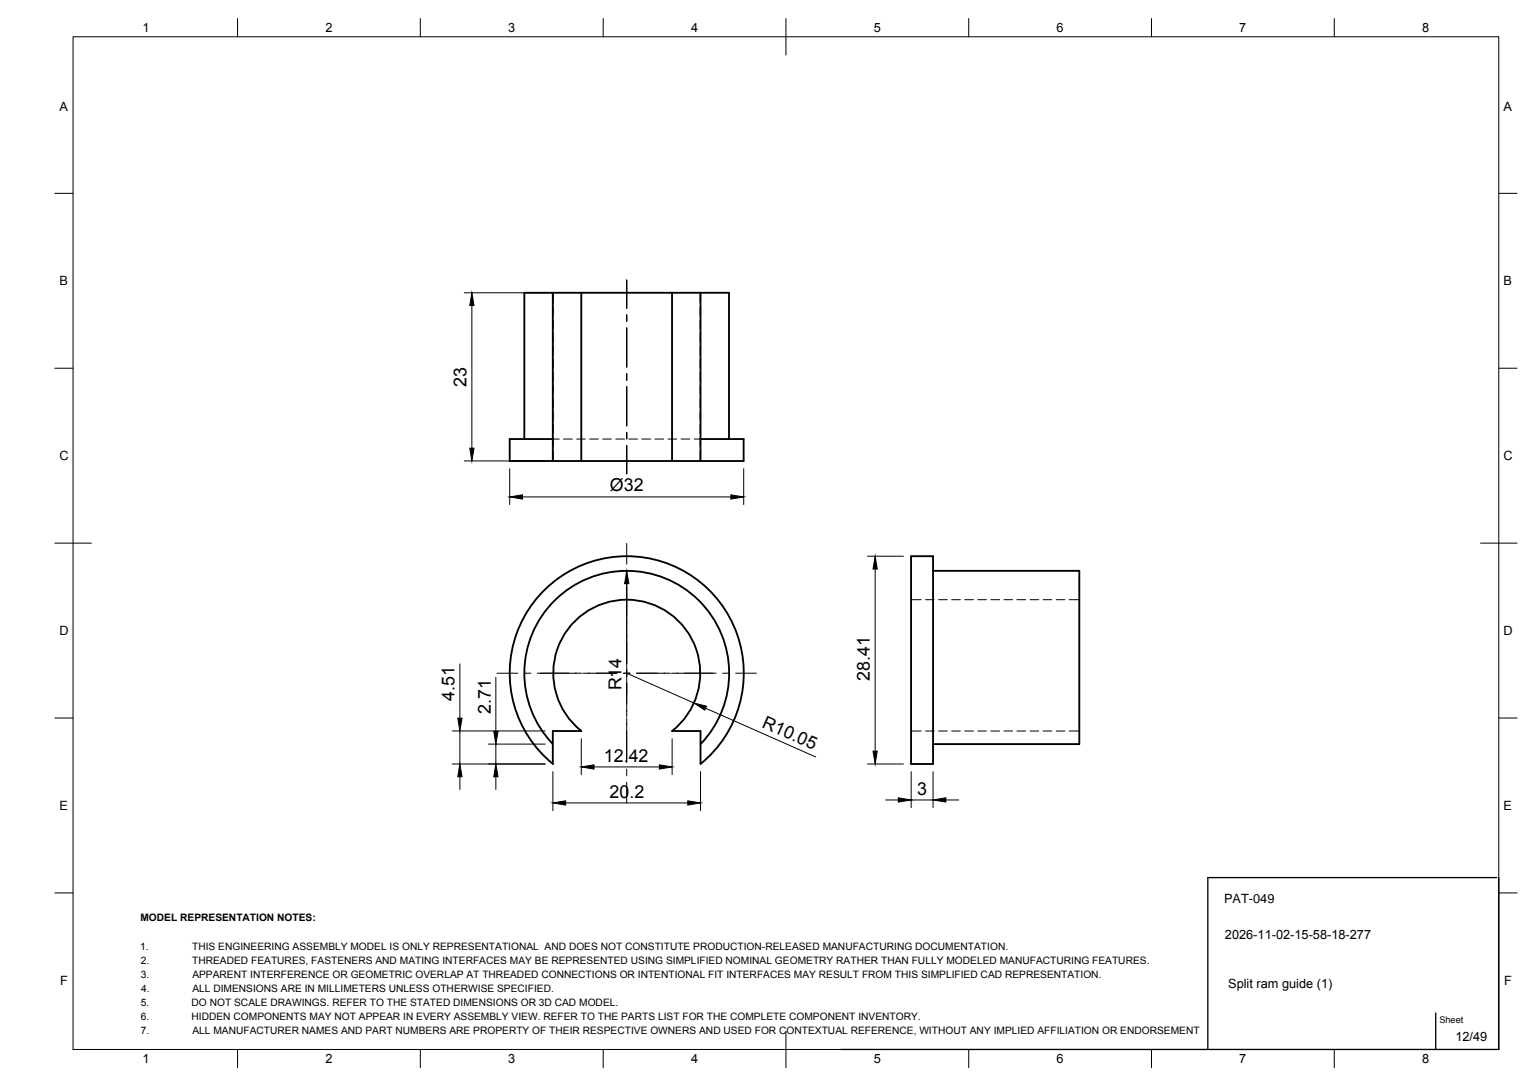
ISO-10303-21;
HEADER;
/* Generated by software containing ST-Developer
 * from STEP Tools, Inc. (www.steptools.com) 
 */

FILE_DESCRIPTION(
/* description */ ('Hand drill press frame (manual)'),
/* implementation_level */ '2;1');

FILE_NAME(
/* name */ 'Split ram guide (1).step',
/* time_stamp */ '2026-10-28T03:25:28-07:00',
/* author */ (''),
/* organization */ (''),
/* preprocessor_version */ 'ST-DEVELOPER v20.2',
/* originating_system */ 'Autodesk Translation Framework v15.17.0.0',
/* authorisation */ '');

FILE_SCHEMA (('AUTOMOTIVE_DESIGN { 1 0 10303 214 3 1 1 }'));
ENDSEC;

DATA;
#10=MECHANICAL_DESIGN_GEOMETRIC_PRESENTATION_REPRESENTATION('',(#626),#33299);
#536=SHAPE_REPRESENTATION_RELATIONSHIP('SRR','None',#33495,#581);
#581=ADVANCED_BREP_SHAPE_REPRESENTATION('',(#678),#33257);
#626=STYLED_ITEM('',(#33807),#678);
#678=MANIFOLD_SOLID_BREP('Body1',#12644);
#956=PLANE('',#13372);
#957=PLANE('',#13373);
#958=PLANE('',#13374);
#959=PLANE('',#13375);
#960=PLANE('',#13376);
#961=PLANE('',#13383);
#962=PLANE('',#13387);
#1441=FACE_OUTER_BOUND('',#2163,.T.);
#1442=FACE_OUTER_BOUND('',#2164,.T.);
#1443=FACE_OUTER_BOUND('',#2165,.T.);
#1444=FACE_OUTER_BOUND('',#2166,.T.);
#1445=FACE_OUTER_BOUND('',#2167,.T.);
#1446=FACE_OUTER_BOUND('',#2168,.T.);
#1447=FACE_OUTER_BOUND('',#2169,.T.);
#1448=FACE_OUTER_BOUND('',#2170,.T.);
#1449=FACE_OUTER_BOUND('',#2171,.T.);
#1450=FACE_OUTER_BOUND('',#2172,.T.);
#2163=EDGE_LOOP('',(#8907,#8908,#8909,#8910));
#2164=EDGE_LOOP('',(#8911,#8912,#8913,#8914));
#2165=EDGE_LOOP('',(#8915,#8916,#8917,#8918,#8919,#8920));
#2166=EDGE_LOOP('',(#8921,#8922,#8923,#8924,#8925,#8926));
#2167=EDGE_LOOP('',(#8927,#8928,#8929,#8930,#8931,#8932));
#2168=EDGE_LOOP('',(#8933,#8934,#8935,#8936));
#2169=EDGE_LOOP('',(#8937,#8938,#8939,#8940));
#2170=EDGE_LOOP('',(#8941,#8942,#8943,#8944));
#2171=EDGE_LOOP('',(#8945,#8946,#8947,#8948));
#2172=EDGE_LOOP('',(#8949,#8950,#8951,#8952,#8953,#8954));
#3045=LINE('',#18532,#4210);
#3046=LINE('',#18534,#4211);
#3047=LINE('',#18536,#4212);
#3048=LINE('',#18537,#4213);
#3049=LINE('',#18541,#4214);
#3050=LINE('',#18543,#4215);
#3051=LINE('',#18545,#4216);
#3052=LINE('',#18546,#4217);
#3053=LINE('',#18549,#4218);
#3054=LINE('',#18551,#4219);
#3055=LINE('',#18553,#4220);
#3056=LINE('',#18555,#4221);
#3057=LINE('',#18556,#4222);
#3058=LINE('',#18559,#4223);
#3059=LINE('',#18561,#4224);
#3060=LINE('',#18563,#4225);
#3061=LINE('',#18565,#4226);
#3062=LINE('',#18566,#4227);
#4210=VECTOR('',#14898,1.);
#4211=VECTOR('',#14899,1.);
#4212=VECTOR('',#14900,1.);
#4213=VECTOR('',#14901,1.);
#4214=VECTOR('',#14904,1.);
#4215=VECTOR('',#14905,1.);
#4216=VECTOR('',#14906,1.);
#4217=VECTOR('',#14907,1.);
#4218=VECTOR('',#14910,1.);
#4219=VECTOR('',#14911,1.);
#4220=VECTOR('',#14912,1.);
#4221=VECTOR('',#14913,1.);
#4222=VECTOR('',#14914,1.);
#4223=VECTOR('',#14917,1.);
#4224=VECTOR('',#14918,1.);
#4225=VECTOR('',#14919,1.);
#4226=VECTOR('',#14920,1.);
#4227=VECTOR('',#14921,1.);
#5286=CIRCLE('',#13377,1.4);
#5287=CIRCLE('',#13378,1.005);
#5288=CIRCLE('',#13380,1.005);
#5289=CIRCLE('',#13382,1.4);
#5290=CIRCLE('',#13384,1.6);
#5291=CIRCLE('',#13386,1.6);
#5775=VERTEX_POINT('',#18530);
#5776=VERTEX_POINT('',#18531);
#5777=VERTEX_POINT('',#18533);
#5778=VERTEX_POINT('',#18535);
#5779=VERTEX_POINT('',#18539);
#5780=VERTEX_POINT('',#18540);
#5781=VERTEX_POINT('',#18542);
#5782=VERTEX_POINT('',#18544);
#5783=VERTEX_POINT('',#18548);
#5784=VERTEX_POINT('',#18550);
#5785=VERTEX_POINT('',#18552);
#5786=VERTEX_POINT('',#18554);
#5787=VERTEX_POINT('',#18558);
#5788=VERTEX_POINT('',#18560);
#5789=VERTEX_POINT('',#18562);
#5790=VERTEX_POINT('',#18564);
#6982=EDGE_CURVE('',#5775,#5776,#3045,.T.);
#6983=EDGE_CURVE('',#5775,#5777,#3046,.T.);
#6984=EDGE_CURVE('',#5778,#5777,#3047,.T.);
#6985=EDGE_CURVE('',#5776,#5778,#3048,.T.);
#6986=EDGE_CURVE('',#5779,#5780,#3049,.T.);
#6987=EDGE_CURVE('',#5781,#5779,#3050,.T.);
#6988=EDGE_CURVE('',#5782,#5781,#3051,.T.);
#6989=EDGE_CURVE('',#5780,#5782,#3052,.T.);
#6990=EDGE_CURVE('',#5783,#5779,#3053,.T.);
#6991=EDGE_CURVE('',#5784,#5783,#3054,.T.);
#6992=EDGE_CURVE('',#5785,#5784,#3055,.T.);
#6993=EDGE_CURVE('',#5786,#5785,#3056,.T.);
#6994=EDGE_CURVE('',#5781,#5786,#3057,.T.);
#6995=EDGE_CURVE('',#5787,#5775,#3058,.T.);
#6996=EDGE_CURVE('',#5788,#5787,#3059,.T.);
#6997=EDGE_CURVE('',#5789,#5788,#3060,.T.);
#6998=EDGE_CURVE('',#5790,#5789,#3061,.T.);
#6999=EDGE_CURVE('',#5777,#5790,#3062,.T.);
#7000=EDGE_CURVE('',#5787,#5786,#5286,.T.);
#7001=EDGE_CURVE('',#5782,#5776,#5287,.T.);
#7002=EDGE_CURVE('',#5780,#5778,#5288,.T.);
#7003=EDGE_CURVE('',#5788,#5785,#5289,.T.);
#7004=EDGE_CURVE('',#5789,#5784,#5290,.T.);
#7005=EDGE_CURVE('',#5790,#5783,#5291,.T.);
#8907=ORIENTED_EDGE('',*,*,#6982,.F.);
#8908=ORIENTED_EDGE('',*,*,#6983,.T.);
#8909=ORIENTED_EDGE('',*,*,#6984,.F.);
#8910=ORIENTED_EDGE('',*,*,#6985,.F.);
#8911=ORIENTED_EDGE('',*,*,#6986,.F.);
#8912=ORIENTED_EDGE('',*,*,#6987,.F.);
#8913=ORIENTED_EDGE('',*,*,#6988,.F.);
#8914=ORIENTED_EDGE('',*,*,#6989,.F.);
#8915=ORIENTED_EDGE('',*,*,#6990,.F.);
#8916=ORIENTED_EDGE('',*,*,#6991,.F.);
#8917=ORIENTED_EDGE('',*,*,#6992,.F.);
#8918=ORIENTED_EDGE('',*,*,#6993,.F.);
#8919=ORIENTED_EDGE('',*,*,#6994,.F.);
#8920=ORIENTED_EDGE('',*,*,#6987,.T.);
#8921=ORIENTED_EDGE('',*,*,#6995,.F.);
#8922=ORIENTED_EDGE('',*,*,#6996,.F.);
#8923=ORIENTED_EDGE('',*,*,#6997,.F.);
#8924=ORIENTED_EDGE('',*,*,#6998,.F.);
#8925=ORIENTED_EDGE('',*,*,#6999,.F.);
#8926=ORIENTED_EDGE('',*,*,#6983,.F.);
#8927=ORIENTED_EDGE('',*,*,#6988,.T.);
#8928=ORIENTED_EDGE('',*,*,#6994,.T.);
#8929=ORIENTED_EDGE('',*,*,#7000,.F.);
#8930=ORIENTED_EDGE('',*,*,#6995,.T.);
#8931=ORIENTED_EDGE('',*,*,#6982,.T.);
#8932=ORIENTED_EDGE('',*,*,#7001,.F.);
#8933=ORIENTED_EDGE('',*,*,#6989,.T.);
#8934=ORIENTED_EDGE('',*,*,#7001,.T.);
#8935=ORIENTED_EDGE('',*,*,#6985,.T.);
#8936=ORIENTED_EDGE('',*,*,#7002,.F.);
#8937=ORIENTED_EDGE('',*,*,#6993,.T.);
#8938=ORIENTED_EDGE('',*,*,#7003,.F.);
#8939=ORIENTED_EDGE('',*,*,#6996,.T.);
#8940=ORIENTED_EDGE('',*,*,#7000,.T.);
#8941=ORIENTED_EDGE('',*,*,#6992,.T.);
#8942=ORIENTED_EDGE('',*,*,#7004,.F.);
#8943=ORIENTED_EDGE('',*,*,#6997,.T.);
#8944=ORIENTED_EDGE('',*,*,#7003,.T.);
#8945=ORIENTED_EDGE('',*,*,#6991,.T.);
#8946=ORIENTED_EDGE('',*,*,#7005,.F.);
#8947=ORIENTED_EDGE('',*,*,#6998,.T.);
#8948=ORIENTED_EDGE('',*,*,#7004,.T.);
#8949=ORIENTED_EDGE('',*,*,#6986,.T.);
#8950=ORIENTED_EDGE('',*,*,#7002,.T.);
#8951=ORIENTED_EDGE('',*,*,#6984,.T.);
#8952=ORIENTED_EDGE('',*,*,#6999,.T.);
#8953=ORIENTED_EDGE('',*,*,#7005,.T.);
#8954=ORIENTED_EDGE('',*,*,#6990,.T.);
#11818=CYLINDRICAL_SURFACE('',#13379,1.005);
#11819=CYLINDRICAL_SURFACE('',#13381,1.4);
#11820=CYLINDRICAL_SURFACE('',#13385,1.6);
#12050=ADVANCED_FACE('',(#1441),#956,.F.);
#12051=ADVANCED_FACE('',(#1442),#957,.F.);
#12052=ADVANCED_FACE('',(#1443),#958,.F.);
#12053=ADVANCED_FACE('',(#1444),#959,.F.);
#12054=ADVANCED_FACE('',(#1445),#960,.F.);
#12055=ADVANCED_FACE('',(#1446),#11818,.F.);
#12056=ADVANCED_FACE('',(#1447),#11819,.T.);
#12057=ADVANCED_FACE('',(#1448),#961,.F.);
#12058=ADVANCED_FACE('',(#1449),#11820,.T.);
#12059=ADVANCED_FACE('',(#1450),#962,.T.);
#12644=CLOSED_SHELL('',(#12050,#12051,#12052,#12053,#12054,#12055,#12056,
#12057,#12058,#12059));
#13371=AXIS2_PLACEMENT_3D('',#18528,#14894,#14895);
#13372=AXIS2_PLACEMENT_3D('',#18529,#14896,#14897);
#13373=AXIS2_PLACEMENT_3D('',#18538,#14902,#14903);
#13374=AXIS2_PLACEMENT_3D('',#18547,#14908,#14909);
#13375=AXIS2_PLACEMENT_3D('',#18557,#14915,#14916);
#13376=AXIS2_PLACEMENT_3D('',#18567,#14922,#14923);
#13377=AXIS2_PLACEMENT_3D('',#18568,#14924,#14925);
#13378=AXIS2_PLACEMENT_3D('',#18569,#14926,#14927);
#13379=AXIS2_PLACEMENT_3D('',#18570,#14928,#14929);
#13380=AXIS2_PLACEMENT_3D('',#18571,#14930,#14931);
#13381=AXIS2_PLACEMENT_3D('',#18572,#14932,#14933);
#13382=AXIS2_PLACEMENT_3D('',#18573,#14934,#14935);
#13383=AXIS2_PLACEMENT_3D('',#18574,#14936,#14937);
#13384=AXIS2_PLACEMENT_3D('',#18575,#14938,#14939);
#13385=AXIS2_PLACEMENT_3D('',#18576,#14940,#14941);
#13386=AXIS2_PLACEMENT_3D('',#18577,#14942,#14943);
#13387=AXIS2_PLACEMENT_3D('',#18578,#14944,#14945);
#14894=DIRECTION('axis',(0.,0.,1.));
#14895=DIRECTION('refdir',(1.,0.,0.));
#14896=DIRECTION('center_axis',(1.,0.,0.));
#14897=DIRECTION('ref_axis',(0.,1.,0.));
#14898=DIRECTION('',(0.,1.,0.));
#14899=DIRECTION('',(0.,0.,1.));
#14900=DIRECTION('',(0.,-1.,0.));
#14901=DIRECTION('',(0.,0.,1.));
#14902=DIRECTION('center_axis',(1.,0.,0.));
#14903=DIRECTION('ref_axis',(0.,1.,0.));
#14904=DIRECTION('',(0.,-1.,0.));
#14905=DIRECTION('',(0.,0.,1.));
#14906=DIRECTION('',(0.,1.,0.));
#14907=DIRECTION('',(0.,0.,-1.));
#14908=DIRECTION('center_axis',(0.,1.,0.));
#14909=DIRECTION('ref_axis',(-1.,0.,0.));
#14910=DIRECTION('',(1.,0.,0.));
#14911=DIRECTION('',(0.,0.,1.));
#14912=DIRECTION('',(-1.,0.,0.));
#14913=DIRECTION('',(0.,0.,1.));
#14914=DIRECTION('',(-1.,0.,0.));
#14915=DIRECTION('center_axis',(0.,-1.,0.));
#14916=DIRECTION('ref_axis',(1.,0.,0.));
#14917=DIRECTION('',(1.,0.,0.));
#14918=DIRECTION('',(0.,0.,-1.));
#14919=DIRECTION('',(1.,0.,0.));
#14920=DIRECTION('',(0.,0.,-1.));
#14921=DIRECTION('',(-1.,0.,0.));
#14922=DIRECTION('center_axis',(0.,0.,1.));
#14923=DIRECTION('ref_axis',(1.,0.,0.));
#14924=DIRECTION('center_axis',(0.,0.,1.));
#14925=DIRECTION('ref_axis',(1.,0.,0.));
#14926=DIRECTION('center_axis',(0.,0.,-1.));
#14927=DIRECTION('ref_axis',(1.,0.,0.));
#14928=DIRECTION('center_axis',(0.,0.,1.));
#14929=DIRECTION('ref_axis',(1.,0.,0.));
#14930=DIRECTION('center_axis',(0.,0.,-1.));
#14931=DIRECTION('ref_axis',(1.,0.,0.));
#14932=DIRECTION('center_axis',(0.,0.,1.));
#14933=DIRECTION('ref_axis',(1.,0.,0.));
#14934=DIRECTION('center_axis',(0.,0.,1.));
#14935=DIRECTION('ref_axis',(1.,0.,0.));
#14936=DIRECTION('center_axis',(0.,0.,1.));
#14937=DIRECTION('ref_axis',(1.,0.,0.));
#14938=DIRECTION('center_axis',(0.,0.,1.));
#14939=DIRECTION('ref_axis',(1.,0.,0.));
#14940=DIRECTION('center_axis',(0.,0.,1.));
#14941=DIRECTION('ref_axis',(1.,0.,0.));
#14942=DIRECTION('center_axis',(0.,0.,1.));
#14943=DIRECTION('ref_axis',(1.,0.,0.));
#14944=DIRECTION('center_axis',(0.,0.,1.));
#14945=DIRECTION('ref_axis',(1.,0.,0.));
#18528=CARTESIAN_POINT('',(0.,0.,0.));
#18529=CARTESIAN_POINT('Origin',(0.21,-1.01,22.9));
#18530=CARTESIAN_POINT('',(0.21,-1.01,23.));
#18531=CARTESIAN_POINT('',(0.21,-0.621228621362538,23.));
#18532=CARTESIAN_POINT('',(0.21,-0.505,23.));
#18533=CARTESIAN_POINT('',(0.21,-1.01,25.3));
#18534=CARTESIAN_POINT('',(0.21,-1.01,22.9));
#18535=CARTESIAN_POINT('',(0.21,-0.621228621362538,25.3));
#18536=CARTESIAN_POINT('',(0.21,-0.505,25.3));
#18537=CARTESIAN_POINT('',(0.21,-0.621228621362538,23.));
#18538=CARTESIAN_POINT('Origin',(0.21,-1.01,22.9));
#18539=CARTESIAN_POINT('',(0.21,1.01,25.3));
#18540=CARTESIAN_POINT('',(0.21,0.621228621362538,25.3));
#18541=CARTESIAN_POINT('',(0.21,-0.505,25.3));
#18542=CARTESIAN_POINT('',(0.21,1.01,23.));
#18543=CARTESIAN_POINT('',(0.21,1.01,22.9));
#18544=CARTESIAN_POINT('',(0.21,0.621228621362538,23.));
#18545=CARTESIAN_POINT('',(0.21,-0.505,23.));
#18546=CARTESIAN_POINT('',(0.21,0.621228621362538,23.));
#18547=CARTESIAN_POINT('Origin',(0.21,1.01,22.9));
#18548=CARTESIAN_POINT('',(-0.240927072796786,1.01,25.3));
#18549=CARTESIAN_POINT('',(0.605,1.01,25.3));
#18550=CARTESIAN_POINT('',(-0.240927072796786,1.01,25.));
#18551=CARTESIAN_POINT('',(-0.240927072796786,1.01,25.));
#18552=CARTESIAN_POINT('',(0.0305156009506911,1.01,25.));
#18553=CARTESIAN_POINT('',(0.605,1.01,25.));
#18554=CARTESIAN_POINT('',(0.0305156009506911,1.01,23.));
#18555=CARTESIAN_POINT('',(0.0305156009506911,1.01,23.));
#18556=CARTESIAN_POINT('',(0.605,1.01,23.));
#18557=CARTESIAN_POINT('Origin',(-0.7,-1.01,22.9));
#18558=CARTESIAN_POINT('',(0.0305156009506911,-1.01,23.));
#18559=CARTESIAN_POINT('',(0.15,-1.01,23.));
#18560=CARTESIAN_POINT('',(0.0305156009506911,-1.01,25.));
#18561=CARTESIAN_POINT('',(0.0305156009506911,-1.01,23.));
#18562=CARTESIAN_POINT('',(-0.240927072796786,-1.01,25.));
#18563=CARTESIAN_POINT('',(0.15,-1.01,25.));
#18564=CARTESIAN_POINT('',(-0.240927072796786,-1.01,25.3));
#18565=CARTESIAN_POINT('',(-0.240927072796786,-1.01,25.));
#18566=CARTESIAN_POINT('',(0.15,-1.01,25.3));
#18567=CARTESIAN_POINT('Origin',(1.,0.,23.));
#18568=CARTESIAN_POINT('Origin',(1.,0.,23.));
#18569=CARTESIAN_POINT('Origin',(1.,0.,23.));
#18570=CARTESIAN_POINT('Origin',(1.,0.,23.));
#18571=CARTESIAN_POINT('Origin',(1.,0.,25.3));
#18572=CARTESIAN_POINT('Origin',(1.,0.,23.));
#18573=CARTESIAN_POINT('Origin',(1.,0.,25.));
#18574=CARTESIAN_POINT('Origin',(1.,0.,25.));
#18575=CARTESIAN_POINT('Origin',(1.,0.,25.));
#18576=CARTESIAN_POINT('Origin',(1.,0.,25.));
#18577=CARTESIAN_POINT('Origin',(1.,0.,25.3));
#18578=CARTESIAN_POINT('Origin',(1.,0.,25.3));
#33205=UNCERTAINTY_MEASURE_WITH_UNIT(LENGTH_MEASURE(0.001),#33300,
'DISTANCE_ACCURACY_VALUE',
'Maximum model space distance between geometric entities at asserted c
onnectivities');
#33247=UNCERTAINTY_MEASURE_WITH_UNIT(LENGTH_MEASURE(0.001),#33300,
'DISTANCE_ACCURACY_VALUE',
'Maximum model space distance between geometric entities at asserted c
onnectivities');
#33257=(
GEOMETRIC_REPRESENTATION_CONTEXT(3)
GLOBAL_UNCERTAINTY_ASSIGNED_CONTEXT((#33205))
GLOBAL_UNIT_ASSIGNED_CONTEXT((#33300,#33302,#33303))
REPRESENTATION_CONTEXT('','3D')
);
#33299=(
GEOMETRIC_REPRESENTATION_CONTEXT(3)
GLOBAL_UNCERTAINTY_ASSIGNED_CONTEXT((#33247))
GLOBAL_UNIT_ASSIGNED_CONTEXT((#33300,#33302,#33303))
REPRESENTATION_CONTEXT('','3D')
);
#33300=(
LENGTH_UNIT()
NAMED_UNIT(*)
SI_UNIT(.CENTI.,.METRE.)
);
#33302=(
NAMED_UNIT(*)
PLANE_ANGLE_UNIT()
SI_UNIT($,.RADIAN.)
);
#33303=(
NAMED_UNIT(*)
SI_UNIT($,.STERADIAN.)
SOLID_ANGLE_UNIT()
);
#33313=SHAPE_DEFINITION_REPRESENTATION(#33364,#33495);
#33364=PRODUCT_DEFINITION_SHAPE('',$,#33547);
#33495=SHAPE_REPRESENTATION('',(#13371),#33257);
#33537=PRODUCT_DEFINITION_CONTEXT('part definition',#33692,'design');
#33547=PRODUCT_DEFINITION('Split ram guide (1)','Split ram guide (1)',#33598,
#33537);
#33598=PRODUCT_DEFINITION_FORMATION('',$,#33703);
#33692=APPLICATION_CONTEXT(
'Core Data for Automotive Mechanical Design Process');
#33693=PRODUCT_CONTEXT('part definition',#33692,'mechanical');
#33703=PRODUCT('Split ram guide (1)','Split ram guide (1)',
'Split ram guide (1)',(#33693));
#33801=COLOUR_RGB('Sky Blue',0.24,0.69,0.87);
#33802=FILL_AREA_STYLE_COLOUR('',#33801);
#33803=FILL_AREA_STYLE('',(#33802));
#33804=SURFACE_STYLE_FILL_AREA(#33803);
#33805=SURFACE_SIDE_STYLE('',(#33804));
#33806=SURFACE_STYLE_USAGE(.BOTH.,#33805);
#33807=PRESENTATION_STYLE_ASSIGNMENT((#33806));
ENDSEC;
END-ISO-10303-21;
